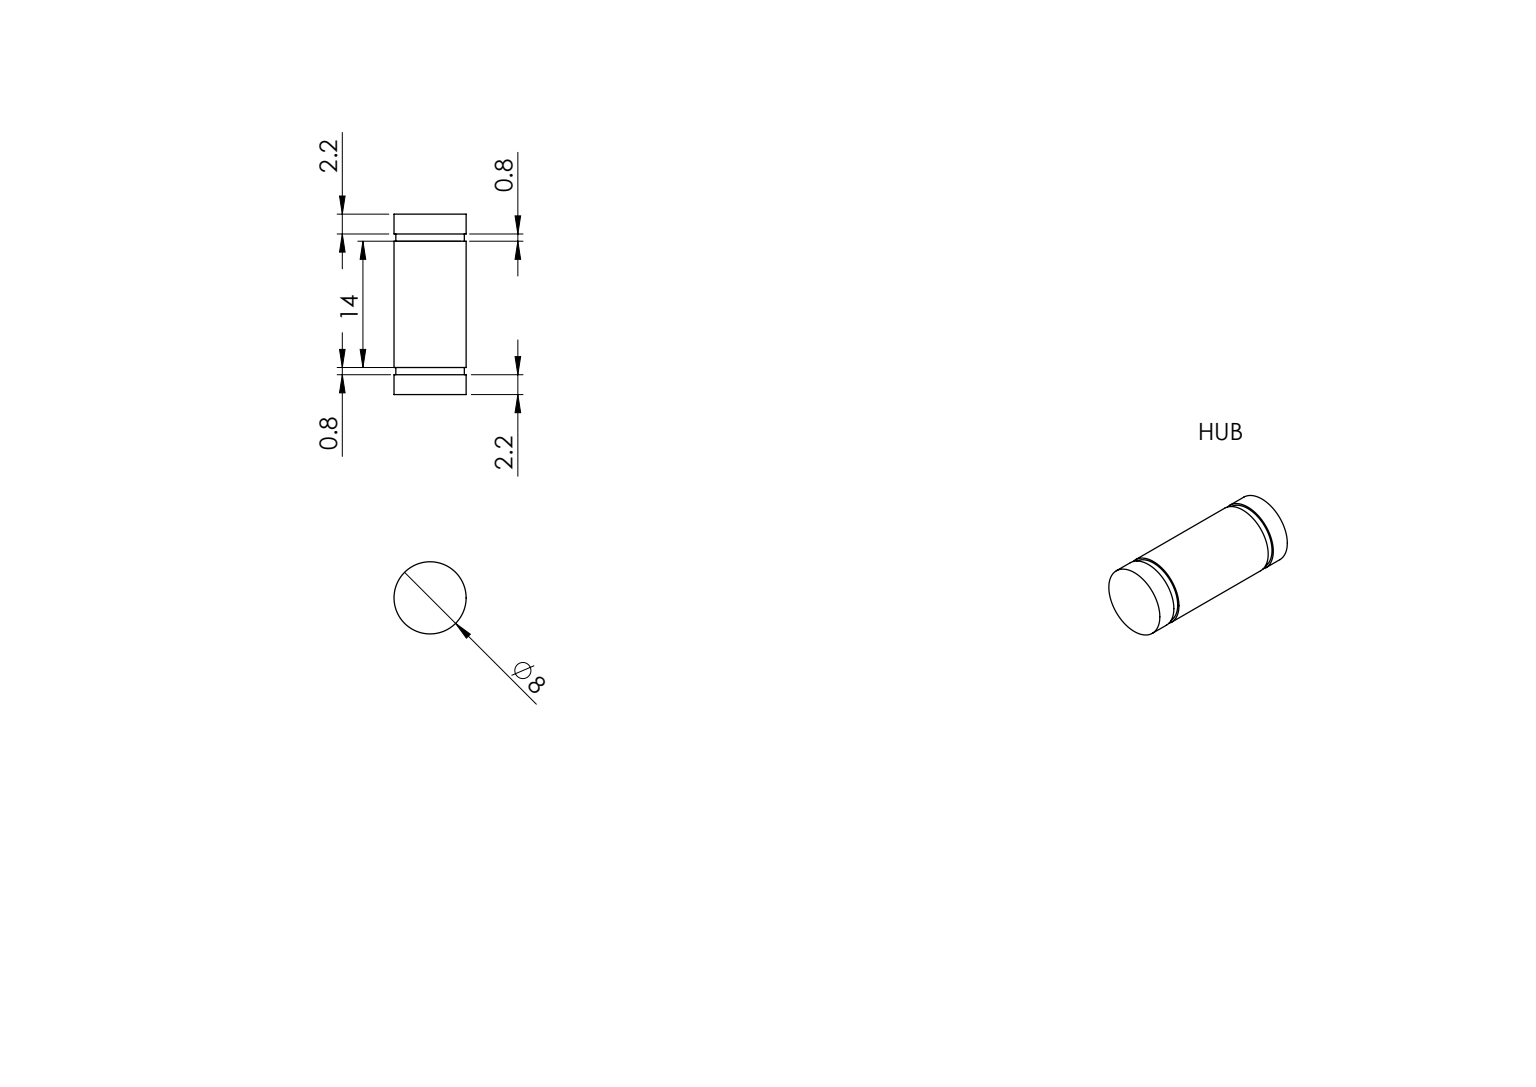
ISO-10303-21;
HEADER;
FILE_DESCRIPTION (('STEP AP214'),
    '1' );
FILE_NAME ('hub.step',
    '2026-10-31T03:41:51',
    ( '' ),
    ( '' ),
    'SwSTEP 2.0',
    'SolidWorks 2026',
    '' );
FILE_SCHEMA (( 'AUTOMOTIVE_DESIGN' ));
ENDSEC;

DATA;
#14=DIRECTION ( 'NONE',  ( -0.9873505073845697533, 0.1585527532634883052, 0.000000000000000000 ) ) ;
#15=CARTESIAN_POINT ( 'NONE',  ( 3.510166481118872639, 1.455586230640303791, -7.000000000000007994 ) ) ;
#136=FACE_BOUND ( 'NONE', #13544, .T. ) ;
#172=AXIS2_PLACEMENT_3D ( 'NONE', #5466, #3375, #833 ) ;
#177=ORIENTED_EDGE ( 'NONE', *, *, #10181, .F. ) ;
#188=VERTEX_POINT ( 'NONE', #5888 ) ;
#271=DIRECTION ( 'NONE',  ( -0.000000000000000000, -0.000000000000000000, -1.000000000000000000 ) ) ;
#281=AXIS2_PLACEMENT_3D ( 'NONE', #6195, #5139, #2580 ) ;
#334=EDGE_LOOP ( 'NONE', ( #5406, #2632 ) ) ;
#361=AXIS2_PLACEMENT_3D ( 'NONE', #2405, #5025, #1550 ) ;
#566=( NAMED_UNIT ( * ) SI_UNIT ( $, .STERADIAN. ) SOLID_ANGLE_UNIT ( ) );
#571=CLOSED_SHELL ( 'NONE', ( #13465, #1305, #9432, #9490, #3541, #14835, #4258, #10117, #4020, #1002, #1343, #9186, #11729, #8337, #8823, #13143 ) ) ;
#577=FACE_OUTER_BOUND ( 'NONE', #11814, .T. ) ;
#591=CIRCLE ( 'NONE', #1085, 3.799999999999999378 ) ;
#602=FACE_BOUND ( 'NONE', #4896, .T. ) ;
#684=ORIENTED_EDGE ( 'NONE', *, *, #14154, .F. ) ;
#686=CARTESIAN_POINT ( 'NONE',  ( 4.000000000000000888, 4.898587196589413815E-16, 10.00000000000000000 ) ) ;
#707=AXIS2_PLACEMENT_3D ( 'NONE', #4857, #13219, #9532 ) ;
#713=CYLINDRICAL_SURFACE ( 'NONE', #1338, 3.799999999999999378 ) ;
#813=CARTESIAN_POINT ( 'NONE',  ( -3.510166481118844661, -1.455586230640303347, -7.000000000000007994 ) ) ;
#833=DIRECTION ( 'NONE',  ( -1.000000000000000000, 0.000000000000000000, 0.000000000000000000 ) ) ;
#883=VERTEX_POINT ( 'NONE', #14448 ) ;
#897=CARTESIAN_POINT ( 'NONE',  ( 3.751931928061364552, -0.6025004624012525456, 7.799999999999990052 ) ) ;
#931=DIRECTION ( 'NONE',  ( 1.000000000000000000, 0.000000000000000000, 0.000000000000000000 ) ) ;
#943=CARTESIAN_POINT ( 'NONE',  ( 1.387778780781445676E-14, 0.000000000000000000, -7.800000000000008704 ) ) ;
#1002=ADVANCED_FACE ( 'NONE', ( #5726 ), #2188, .F. ) ;
#1012=CARTESIAN_POINT ( 'NONE',  ( 0.000000000000000000, 0.000000000000000000, -7.000000000000007994 ) ) ;
#1035=ORIENTED_EDGE ( 'NONE', *, *, #4321, .T. ) ;
#1080=DIRECTION ( 'NONE',  ( -5.339417856040273846E-17, -1.063174570779084847E-17, 1.000000000000000000 ) ) ;
#1085=AXIS2_PLACEMENT_3D ( 'NONE', #14018, #3483, #4499 ) ;
#1134=EDGE_CURVE ( 'NONE', #3521, #6501, #14102, .T. ) ;
#1157=CIRCLE ( 'NONE', #5838, 4.000000000000000888 ) ;
#1171=LINE ( 'NONE', #10842, #10236 ) ;
#1188=AXIS2_PLACEMENT_3D ( 'NONE', #7647, #14417, #6413 ) ;
#1211=EDGE_LOOP ( 'NONE', ( #2408, #10707 ) ) ;
#1233=EDGE_LOOP ( 'NONE', ( #2848, #13553 ) ) ;
#1243=DIRECTION ( 'NONE',  ( -0.000000000000000000, -0.000000000000000000, -1.000000000000000000 ) ) ;
#1305=ADVANCED_FACE ( 'NONE', ( #13545 ), #713, .T. ) ;
#1338=AXIS2_PLACEMENT_3D ( 'NONE', #9790, #10088, #14487 ) ;
#1343=ADVANCED_FACE ( 'NONE', ( #7786, #14944 ), #12543, .T. ) ;
#1376=AXIS2_PLACEMENT_3D ( 'NONE', #7353, #6187, #9640 ) ;
#1550=DIRECTION ( 'NONE',  ( -0.9873505073845698643, 0.1585527532634883330, -5.103307673902845341E-17 ) ) ;
#1569=EDGE_CURVE ( 'NONE', #883, #13931, #1171, .T. ) ;
#1595=CARTESIAN_POINT ( 'NONE',  ( 0.000000000000000000, 0.000000000000000000, 10.00000000000000000 ) ) ;
#1602=VECTOR ( 'NONE', #10196, 1000.000000000000000 ) ;
#1616=LINE ( 'NONE', #686, #9254 ) ;
#1694=DIRECTION ( 'NONE',  ( -5.339417856040273846E-17, -1.063174570779084847E-17, 1.000000000000000000 ) ) ;
#1753=EDGE_LOOP ( 'NONE', ( #13832, #7384, #14688, #11419 ) ) ;
#1802=( NAMED_UNIT ( * ) SI_UNIT ( $, .STERADIAN. ) SOLID_ANGLE_UNIT ( ) );
#1883=( LENGTH_UNIT ( ) NAMED_UNIT ( * ) SI_UNIT ( .MILLI., .METRE. ) );
#1912=CARTESIAN_POINT ( 'NONE',  ( 0.000000000000000000, 0.000000000000000000, 10.00000000000000000 ) ) ;
#1943=DIRECTION ( 'NONE',  ( -5.339417856040273846E-17, -1.063174570779084847E-17, 1.000000000000000000 ) ) ;
#1951=DIRECTION ( 'NONE',  ( -0.000000000000000000, 0.000000000000000000, -1.000000000000000000 ) ) ;
#2008=VERTEX_POINT ( 'NONE', #9753 ) ;
#2018=CARTESIAN_POINT ( 'NONE',  ( 1.387778780781445676E-14, 0.000000000000000000, -7.000000000000007994 ) ) ;
#2034=APPLICATION_CONTEXT ( 'automotive_design' ) ;
#2070=EDGE_CURVE ( 'NONE', #12014, #3521, #14593, .T. ) ;
#2083=FACE_OUTER_BOUND ( 'NONE', #4286, .T. ) ;
#2089=PRODUCT_DEFINITION_FORMATION_WITH_SPECIFIED_SOURCE ( 'ANY', '', #9463, .NOT_KNOWN. ) ;
#2101=CIRCLE ( 'NONE', #8723, 4.000000000000000888 ) ;
#2102=SURFACE_SIDE_STYLE ('',( #8863 ) ) ;
#2116=EDGE_CURVE ( 'NONE', #13784, #883, #8011, .T. ) ;
#2135=MECHANICAL_DESIGN_GEOMETRIC_PRESENTATION_REPRESENTATION('',(#3118),#5350);
#2171=CARTESIAN_POINT ( 'NONE',  ( 4.000000000000000888, 4.898587196589413815E-16, 10.00000000000000000 ) ) ;
#2179=AXIS2_PLACEMENT_3D ( 'NONE', #10380, #2241, #6855 ) ;
#2188=PLANE ( 'NONE',  #4532 ) ;
#2206=DIRECTION ( 'NONE',  ( 1.000000000000000000, 0.000000000000000000, 0.000000000000000000 ) ) ;
#2241=DIRECTION ( 'NONE',  ( 0.000000000000000000, 0.000000000000000000, -1.000000000000000000 ) ) ;
#2256=EDGE_LOOP ( 'NONE', ( #4202, #12754, #1035, #5511 ) ) ;
#2328=AXIS2_PLACEMENT_3D ( 'NONE', #7519, #12342, #12193 ) ;
#2380=AXIS2_PLACEMENT_3D ( 'NONE', #12215, #1694, #6377 ) ;
#2405=CARTESIAN_POINT ( 'NONE',  ( 0.000000000000000000, 3.361026734705063745E-15, 7.799999999999990052 ) ) ;
#2408=ORIENTED_EDGE ( 'NONE', *, *, #10953, .F. ) ;
#2414=CARTESIAN_POINT ( 'NONE',  ( -4.000000000000000888, 0.000000000000000000, 10.00000000000000000 ) ) ;
#2466=ORIENTED_EDGE ( 'NONE', *, *, #8770, .F. ) ;
#2512=EDGE_CURVE ( 'NONE', #12014, #2008, #6927, .T. ) ;
#2514=ORIENTED_EDGE ( 'NONE', *, *, #9096, .T. ) ;
#2517=FACE_OUTER_BOUND ( 'NONE', #8195, .T. ) ;
#2580=DIRECTION ( 'NONE',  ( -0.9873505073845697533, 0.1585527532634883052, 0.000000000000000000 ) ) ;
#2582=CIRCLE ( 'NONE', #6514, 3.799999999999999378 ) ;
#2632=ORIENTED_EDGE ( 'NONE', *, *, #6864, .T. ) ;
#2652=CIRCLE ( 'NONE', #14941, 4.000000000000000888 ) ;
#2658=LINE ( 'NONE', #6929, #4395 ) ;
#2743=EDGE_LOOP ( 'NONE', ( #6165, #4935, #6542, #7775 ) ) ;
#2819=CARTESIAN_POINT ( 'NONE',  ( -3.510166481118844661, -1.455586230640303347, -7.800000000000008704 ) ) ;
#2820=DIRECTION ( 'NONE',  ( -1.000000000000000000, 0.000000000000000000, 0.000000000000000000 ) ) ;
#2839=CYLINDRICAL_SURFACE ( 'NONE', #2380, 3.799999999999999378 ) ;
#2844=DIRECTION ( 'NONE',  ( 5.339417856040273846E-17, 1.063174570779084847E-17, -1.000000000000000000 ) ) ;
#2848=ORIENTED_EDGE ( 'NONE', *, *, #8770, .T. ) ;
#2906=PRODUCT_CONTEXT ( 'NONE', #2917, 'mechanical' ) ;
#2917=APPLICATION_CONTEXT ( 'automotive_design' ) ;
#2955=CARTESIAN_POINT ( 'NONE',  ( 3.510166481118872639, 1.455586230640303791, -7.000000000000007994 ) ) ;
#3031=PRESENTATION_STYLE_ASSIGNMENT (( #7803 ) ) ;
#3071=DIRECTION ( 'NONE',  ( 1.000000000000000000, 0.000000000000000000, 0.000000000000000000 ) ) ;
#3118=STYLED_ITEM('',(#15286),#3717);
#3147=CIRCLE ( 'NONE', #12705, 4.000000000000000888 ) ;
#3150=CARTESIAN_POINT ( 'NONE',  ( 3.751931928061364552, -0.6025004624012525456, 6.999999999999989342 ) ) ;
#3197=EDGE_CURVE ( 'NONE', #13784, #6657, #10149, .T. ) ;
#3243=ORIENTED_EDGE ( 'NONE', *, *, #7762, .F. ) ;
#3346=VERTEX_POINT ( 'NONE', #7605 ) ;
#3375=DIRECTION ( 'NONE',  ( -0.000000000000000000, -0.000000000000000000, -1.000000000000000000 ) ) ;
#3421=CARTESIAN_POINT ( 'NONE',  ( 0.000000000000000000, 0.000000000000000000, 10.00000000000000000 ) ) ;
#3483=DIRECTION ( 'NONE',  ( 5.339417856040273846E-17, 1.063174570779084847E-17, -1.000000000000000000 ) ) ;
#3501=ORIENTED_EDGE ( 'NONE', *, *, #3197, .T. ) ;
#3521=VERTEX_POINT ( 'NONE', #897 ) ;
#3541=ADVANCED_FACE ( 'NONE', ( #7749 ), #6821, .T. ) ;
#3551=CARTESIAN_POINT ( 'NONE',  ( 1.387778780781445676E-14, 0.000000000000000000, -7.000000000000007994 ) ) ;
#3604=AXIS2_PLACEMENT_3D ( 'NONE', #12463, #1080, #5778 ) ;
#3615=AXIS2_PLACEMENT_3D ( 'NONE', #5465, #4381, #3071 ) ;
#3618=AXIS2_PLACEMENT_3D ( 'NONE', #11876, #271, #10525 ) ;
#3630=DIRECTION ( 'NONE',  ( 0.000000000000000000, 0.000000000000000000, 1.000000000000000000 ) ) ;
#3717=MANIFOLD_SOLID_BREP ( 'Mirror2', #571 ) ;
#3797=CIRCLE ( 'NONE', #5048, 4.000000000000000888 ) ;
#3798=CYLINDRICAL_SURFACE ( 'NONE', #1188, 4.000000000000000888 ) ;
#3818=CARTESIAN_POINT ( 'NONE',  ( 0.000000000000000000, 0.000000000000000000, 7.799999999999990052 ) ) ;
#3932=CIRCLE ( 'NONE', #9806, 4.000000000000000888 ) ;
#3946=UNCERTAINTY_MEASURE_WITH_UNIT (LENGTH_MEASURE( 1.000000000000000082E-05 ), #1883, 'distance_accuracy_value', 'NONE');
#3986=DIRECTION ( 'NONE',  ( -1.000000000000000000, 0.000000000000000000, 0.000000000000000000 ) ) ;
#4020=ADVANCED_FACE ( 'NONE', ( #10493 ), #15108, .T. ) ;
#4202=ORIENTED_EDGE ( 'NONE', *, *, #11610, .F. ) ;
#4258=ADVANCED_FACE ( 'NONE', ( #11161 ), #7709, .T. ) ;
#4276=VERTEX_POINT ( 'NONE', #11317 ) ;
#4286=EDGE_LOOP ( 'NONE', ( #12799, #3243, #14483, #11996 ) ) ;
#4300=CYLINDRICAL_SURFACE ( 'NONE', #172, 4.000000000000000888 ) ;
#4321=EDGE_CURVE ( 'NONE', #10385, #9762, #9622, .T. ) ;
#4381=DIRECTION ( 'NONE',  ( -5.339417856040273846E-17, -1.063174570779084847E-17, 1.000000000000000000 ) ) ;
#4395=VECTOR ( 'NONE', #8941, 1000.000000000000000 ) ;
#4499=DIRECTION ( 'NONE',  ( -0.9873505073845697533, 0.1585527532634883052, 0.000000000000000000 ) ) ;
#4532=AXIS2_PLACEMENT_3D ( 'NONE', #14674, #8966, #9974 ) ;
#4583=( GEOMETRIC_REPRESENTATION_CONTEXT ( 3 ) GLOBAL_UNCERTAINTY_ASSIGNED_CONTEXT ( ( #3946 ) ) GLOBAL_UNIT_ASSIGNED_CONTEXT ( ( #1883, #12487, #10101 ) ) REPRESENTATION_CONTEXT ( 'NONE', 'WORKASPACE' ) );
#4633=ORIENTED_EDGE ( 'NONE', *, *, #14894, .T. ) ;
#4673=DIRECTION ( 'NONE',  ( -0.9237280213470681067, -0.3830490080632377725, 0.000000000000000000 ) ) ;
#4700=ORIENTED_EDGE ( 'NONE', *, *, #1134, .F. ) ;
#4722=ORIENTED_EDGE ( 'NONE', *, *, #8548, .F. ) ;
#4857=CARTESIAN_POINT ( 'NONE',  ( 1.387778780781445676E-14, 0.000000000000000000, -7.800000000000008704 ) ) ;
#4871=ORIENTED_EDGE ( 'NONE', *, *, #6559, .T. ) ;
#4896=EDGE_LOOP ( 'NONE', ( #14625, #8838 ) ) ;
#4935=ORIENTED_EDGE ( 'NONE', *, *, #2070, .T. ) ;
#4954=CARTESIAN_POINT ( 'NONE',  ( 4.000000000000000888, 4.898587196589413815E-16, -10.00000000000000000 ) ) ;
#5025=DIRECTION ( 'NONE',  ( -5.339417856040274462E-17, -1.063174570779084693E-17, 1.000000000000000000 ) ) ;
#5048=AXIS2_PLACEMENT_3D ( 'NONE', #1595, #5741, #2206 ) ;
#5139=DIRECTION ( 'NONE',  ( 5.339417856040273846E-17, 1.063174570779084847E-17, -1.000000000000000000 ) ) ;
#5164=ORIENTED_EDGE ( 'NONE', *, *, #5328, .F. ) ;
#5180=ORIENTED_EDGE ( 'NONE', *, *, #10953, .T. ) ;
#5220=CARTESIAN_POINT ( 'NONE',  ( 0.000000000000000000, 0.000000000000000000, 10.00000000000000000 ) ) ;
#5271=CARTESIAN_POINT ( 'NONE',  ( 4.000000000000000888, 4.898587196589413815E-16, 6.999999999999989342 ) ) ;
#5283=VECTOR ( 'NONE', #8994, 1000.000000000000000 ) ;
#5292=AXIS2_PLACEMENT_3D ( 'NONE', #10991, #2844, #12130 ) ;
#5296=CYLINDRICAL_SURFACE ( 'NONE', #14910, 4.000000000000000888 ) ;
#5316=AXIS2_PLACEMENT_3D ( 'NONE', #12069, #11998, #8688 ) ;
#5321=PLANE ( 'NONE',  #14351 ) ;
#5328=EDGE_CURVE ( 'NONE', #14141, #11359, #3932, .T. ) ;
#5333=VERTEX_POINT ( 'NONE', #13616 ) ;
#5350=( GEOMETRIC_REPRESENTATION_CONTEXT ( 3 ) GLOBAL_UNCERTAINTY_ASSIGNED_CONTEXT ( ( #13840 ) ) GLOBAL_UNIT_ASSIGNED_CONTEXT ( ( #6421, #11104, #566 ) ) REPRESENTATION_CONTEXT ( 'NONE', 'WORKASPACE' ) );
#5406=ORIENTED_EDGE ( 'NONE', *, *, #11003, .T. ) ;
#5412=EDGE_LOOP ( 'NONE', ( #684, #14580, #13715, #9552 ) ) ;
#5465=CARTESIAN_POINT ( 'NONE',  ( 0.000000000000000000, 0.000000000000000000, 6.999999999999989342 ) ) ;
#5466=CARTESIAN_POINT ( 'NONE',  ( 0.000000000000000000, 0.000000000000000000, 10.00000000000000000 ) ) ;
#5469=CARTESIAN_POINT ( 'NONE',  ( 4.271534284832219323E-17, 3.369532131271296443E-15, 6.999999999999989342 ) ) ;
#5500=SHAPE_REPRESENTATION_RELATIONSHIP ( 'NONE' , 'NONE' ,  #5737, #14983 ) ;
#5511=ORIENTED_EDGE ( 'NONE', *, *, #11130, .F. ) ;
#5567=DIRECTION ( 'NONE',  ( -0.000000000000000000, -0.000000000000000000, -1.000000000000000000 ) ) ;
#5580=AXIS2_PLACEMENT_3D ( 'NONE', #1912, #10350, #6604 ) ;
#5650=EDGE_LOOP ( 'NONE', ( #5180, #3501, #4633, #6543 ) ) ;
#5726=FACE_OUTER_BOUND ( 'NONE', #7587, .T. ) ;
#5737=SHAPE_REPRESENTATION ( 'hub', ( #1376 ), #12207 ) ;
#5741=DIRECTION ( 'NONE',  ( 0.000000000000000000, 0.000000000000000000, 1.000000000000000000 ) ) ;
#5778=DIRECTION ( 'NONE',  ( -0.9873505073845697533, 0.1585527532634883052, 0.000000000000000000 ) ) ;
#5805=VECTOR ( 'NONE', #14677, 1000.000000000000000 ) ;
#5838=AXIS2_PLACEMENT_3D ( 'NONE', #10962, #13505, #7662 ) ;
#5888=CARTESIAN_POINT ( 'NONE',  ( -4.000000000000000888, 0.000000000000000000, 10.00000000000000000 ) ) ;
#5946=DIRECTION ( 'NONE',  ( -0.000000000000000000, -0.000000000000000000, -1.000000000000000000 ) ) ;
#5953=AXIS2_PLACEMENT_3D ( 'NONE', #943, #12395, #10321 ) ;
#6018=CIRCLE ( 'NONE', #12873, 3.799999999999999378 ) ;
#6069=CIRCLE ( 'NONE', #7550, 4.000000000000000888 ) ;
#6091=DIRECTION ( 'NONE',  ( 1.000000000000000000, 0.000000000000000000, 0.000000000000000000 ) ) ;
#6162=CARTESIAN_POINT ( 'NONE',  ( 0.000000000000000000, 0.000000000000000000, -10.00000000000000000 ) ) ;
#6165=ORIENTED_EDGE ( 'NONE', *, *, #2512, .F. ) ;
#6187=DIRECTION ( 'NONE',  ( 0.000000000000000000, 0.000000000000000000, 1.000000000000000000 ) ) ;
#6195=CARTESIAN_POINT ( 'NONE',  ( 4.271534284832219323E-17, 3.369532131271296443E-15, 6.999999999999989342 ) ) ;
#6203=ORIENTED_EDGE ( 'NONE', *, *, #14886, .F. ) ;
#6235=FACE_BOUND ( 'NONE', #13768, .T. ) ;
#6294=ORIENTED_EDGE ( 'NONE', *, *, #5328, .T. ) ;
#6377=DIRECTION ( 'NONE',  ( -0.9873505073845697533, 0.1585527532634883052, 0.000000000000000000 ) ) ;
#6413=DIRECTION ( 'NONE',  ( -1.000000000000000000, 0.000000000000000000, 0.000000000000000000 ) ) ;
#6421=( LENGTH_UNIT ( ) NAMED_UNIT ( * ) SI_UNIT ( .MILLI., .METRE. ) );
#6501=VERTEX_POINT ( 'NONE', #11698 ) ;
#6514=AXIS2_PLACEMENT_3D ( 'NONE', #3551, #3630, #8320 ) ;
#6540=VERTEX_POINT ( 'NONE', #15 ) ;
#6542=ORIENTED_EDGE ( 'NONE', *, *, #1134, .T. ) ;
#6543=ORIENTED_EDGE ( 'NONE', *, *, #1569, .F. ) ;
#6559=EDGE_CURVE ( 'NONE', #188, #3346, #15029, .T. ) ;
#6562=CARTESIAN_POINT ( 'NONE',  ( 0.000000000000000000, 0.000000000000000000, 10.00000000000000000 ) ) ;
#6604=DIRECTION ( 'NONE',  ( -1.000000000000000000, 0.000000000000000000, 0.000000000000000000 ) ) ;
#6657=VERTEX_POINT ( 'NONE', #4954 ) ;
#6693=CARTESIAN_POINT ( 'NONE',  ( 4.000000000000000888, 4.898587196589413815E-16, 10.00000000000000000 ) ) ;
#6744=CIRCLE ( 'NONE', #2328, 4.000000000000000888 ) ;
#6747=AXIS2_PLACEMENT_3D ( 'NONE', #13065, #7251, #14 ) ;
#6793=( NAMED_UNIT ( * ) PLANE_ANGLE_UNIT ( ) SI_UNIT ( $, .RADIAN. ) );
#6814=AXIS2_PLACEMENT_3D ( 'NONE', #9407, #14261, #4673 ) ;
#6821=CYLINDRICAL_SURFACE ( 'NONE', #5580, 4.000000000000000888 ) ;
#6855=DIRECTION ( 'NONE',  ( -1.000000000000000000, 0.000000000000000000, 0.000000000000000000 ) ) ;
#6856=DIRECTION ( 'NONE',  ( -0.000000000000000000, -0.000000000000000000, -1.000000000000000000 ) ) ;
#6864=EDGE_CURVE ( 'NONE', #5333, #188, #2652, .T. ) ;
#6927=CIRCLE ( 'NONE', #281, 3.799999999999999378 ) ;
#6929=CARTESIAN_POINT ( 'NONE',  ( -4.000000000000000888, 0.000000000000000000, 10.00000000000000000 ) ) ;
#7055=CIRCLE ( 'NONE', #6814, 3.799999999999999378 ) ;
#7162=ORIENTED_EDGE ( 'NONE', *, *, #12918, .F. ) ;
#7251=DIRECTION ( 'NONE',  ( 5.339417856040273846E-17, 1.063174570779084847E-17, -1.000000000000000000 ) ) ;
#7280=EDGE_LOOP ( 'NONE', ( #6203, #11454 ) ) ;
#7283=CYLINDRICAL_SURFACE ( 'NONE', #3618, 4.000000000000000888 ) ;
#7334=CYLINDRICAL_SURFACE ( 'NONE', #5316, 3.799999999999999378 ) ;
#7353=CARTESIAN_POINT ( 'NONE',  ( 0.000000000000000000, 0.000000000000000000, 0.000000000000000000 ) ) ;
#7384=ORIENTED_EDGE ( 'NONE', *, *, #2116, .T. ) ;
#7403=PLANE ( 'NONE',  #361 ) ;
#7496=CARTESIAN_POINT ( 'NONE',  ( -4.000000000000000888, 0.000000000000000000, -7.000000000000007994 ) ) ;
#7518=DIRECTION ( 'NONE',  ( -5.339417856040273846E-17, -1.063174570779084847E-17, 1.000000000000000000 ) ) ;
#7519=CARTESIAN_POINT ( 'NONE',  ( 0.000000000000000000, 0.000000000000000000, -7.800000000000010481 ) ) ;
#7531=ORIENTED_EDGE ( 'NONE', *, *, #14259, .T. ) ;
#7550=AXIS2_PLACEMENT_3D ( 'NONE', #3818, #7518, #14516 ) ;
#7558=STYLED_ITEM ( 'NONE', ( #3031 ), #14983 ) ;
#7587=EDGE_LOOP ( 'NONE', ( #7162, #14662 ) ) ;
#7605=CARTESIAN_POINT ( 'NONE',  ( -4.000000000000000888, 2.270693314922320170E-33, 7.799999999999990052 ) ) ;
#7647=CARTESIAN_POINT ( 'NONE',  ( 0.000000000000000000, 0.000000000000000000, 10.00000000000000000 ) ) ;
#7662=DIRECTION ( 'NONE',  ( 1.000000000000000000, 0.000000000000000000, 0.000000000000000000 ) ) ;
#7709=CYLINDRICAL_SURFACE ( 'NONE', #10365, 4.000000000000000888 ) ;
#7749=FACE_OUTER_BOUND ( 'NONE', #14904, .T. ) ;
#7762=EDGE_CURVE ( 'NONE', #2008, #12014, #591, .T. ) ;
#7771=PRODUCT_DEFINITION ( 'UNKNOWN', '', #2089, #13466 ) ;
#7775=ORIENTED_EDGE ( 'NONE', *, *, #8037, .F. ) ;
#7786=FACE_BOUND ( 'NONE', #1233, .T. ) ;
#7789=CARTESIAN_POINT ( 'NONE',  ( -3.751931928061364552, 0.6025004624012588739, 6.999999999999989342 ) ) ;
#7803=SURFACE_STYLE_USAGE ( .BOTH. , #2102 ) ;
#7869=CARTESIAN_POINT ( 'NONE',  ( -4.000000000000000888, 2.270693314922320170E-33, 6.999999999999989342 ) ) ;
#7908=CARTESIAN_POINT ( 'NONE',  ( -3.510166481118844661, -1.455586230640303347, -7.000000000000007994 ) ) ;
#7928=CYLINDRICAL_SURFACE ( 'NONE', #3604, 3.799999999999999378 ) ;
#7930=CARTESIAN_POINT ( 'NONE',  ( 0.000000000000000000, 0.000000000000000000, 7.799999999999990052 ) ) ;
#7934=DIRECTION ( 'NONE',  ( -0.9237280213470682178, -0.3830490080632377725, 0.000000000000000000 ) ) ;
#7983=VERTEX_POINT ( 'NONE', #7869 ) ;
#8011=CIRCLE ( 'NONE', #12169, 4.000000000000000888 ) ;
#8037=EDGE_CURVE ( 'NONE', #2008, #6501, #10164, .T. ) ;
#8155=EDGE_LOOP ( 'NONE', ( #4722, #2466, #9128, #15107 ) ) ;
#8167=AXIS2_PLACEMENT_3D ( 'NONE', #3421, #11781, #9400 ) ;
#8169=EDGE_CURVE ( 'NONE', #6501, #3521, #8449, .T. ) ;
#8195=EDGE_LOOP ( 'NONE', ( #11263, #12072, #5164, #177 ) ) ;
#8320=DIRECTION ( 'NONE',  ( -0.9237280213470681067, -0.3830490080632377725, 0.000000000000000000 ) ) ;
#8337=ADVANCED_FACE ( 'NONE', ( #602, #8907 ), #5321, .T. ) ;
#8378=DIRECTION ( 'NONE',  ( 0.000000000000000000, 0.000000000000000000, 1.000000000000000000 ) ) ;
#8449=CIRCLE ( 'NONE', #5292, 3.799999999999999378 ) ;
#8528=PLANE ( 'NONE',  #707 ) ;
#8545=FACE_OUTER_BOUND ( 'NONE', #7280, .T. ) ;
#8548=EDGE_CURVE ( 'NONE', #6540, #10385, #14791, .T. ) ;
#8556=VECTOR ( 'NONE', #5946, 1000.000000000000000 ) ;
#8585=DIRECTION ( 'NONE',  ( -0.000000000000000000, -0.000000000000000000, -1.000000000000000000 ) ) ;
#8688=DIRECTION ( 'NONE',  ( -0.9237280213470681067, -0.3830490080632377725, 0.000000000000000000 ) ) ;
#8693=CARTESIAN_POINT ( 'NONE',  ( 0.000000000000000000, 0.000000000000000000, 10.00000000000000000 ) ) ;
#8723=AXIS2_PLACEMENT_3D ( 'NONE', #6162, #8378, #6091 ) ;
#8770=EDGE_CURVE ( 'NONE', #11997, #6540, #6018, .T. ) ;
#8823=ADVANCED_FACE ( 'NONE', ( #8545, #6235 ), #7403, .F. ) ;
#8838=ORIENTED_EDGE ( 'NONE', *, *, #2512, .T. ) ;
#8854=DIRECTION ( 'NONE',  ( -5.339417856040273846E-17, -1.063174570779084847E-17, 1.000000000000000000 ) ) ;
#8863=SURFACE_STYLE_FILL_AREA ( #11324 ) ;
#8907=FACE_OUTER_BOUND ( 'NONE', #11914, .T. ) ;
#8941=DIRECTION ( 'NONE',  ( -0.000000000000000000, -0.000000000000000000, -1.000000000000000000 ) ) ;
#8966=DIRECTION ( 'NONE',  ( 0.000000000000000000, 0.000000000000000000, 1.000000000000000000 ) ) ;
#8994=DIRECTION ( 'NONE',  ( -0.000000000000000000, -0.000000000000000000, -1.000000000000000000 ) ) ;
#9031=VECTOR ( 'NONE', #6856, 1000.000000000000000 ) ;
#9038=ORIENTED_EDGE ( 'NONE', *, *, #11003, .F. ) ;
#9088=DIRECTION ( 'NONE',  ( -5.339417856040273846E-17, -1.063174570779084847E-17, 1.000000000000000000 ) ) ;
#9096=EDGE_CURVE ( 'NONE', #11359, #14141, #11463, .T. ) ;
#9128=ORIENTED_EDGE ( 'NONE', *, *, #11130, .T. ) ;
#9186=ADVANCED_FACE ( 'NONE', ( #10684, #136 ), #8528, .F. ) ;
#9253=ORIENTED_EDGE ( 'NONE', *, *, #6864, .F. ) ;
#9254=VECTOR ( 'NONE', #12358, 1000.000000000000000 ) ;
#9327=CARTESIAN_POINT ( 'NONE',  ( 1.387778780781445676E-14, 0.000000000000000000, -7.000000000000007994 ) ) ;
#9400=DIRECTION ( 'NONE',  ( 1.000000000000000000, 0.000000000000000000, -0.000000000000000000 ) ) ;
#9407=CARTESIAN_POINT ( 'NONE',  ( 1.387778780781445676E-14, 0.000000000000000000, -7.800000000000008704 ) ) ;
#9432=ADVANCED_FACE ( 'NONE', ( #15058 ), #4300, .T. ) ;
#9463=PRODUCT ( 'hub', 'hub', '', ( #2906 ) ) ;
#9490=ADVANCED_FACE ( 'NONE', ( #2517 ), #7283, .T. ) ;
#9532=DIRECTION ( 'NONE',  ( -0.9237280213470682178, -0.3830490080632377725, 0.000000000000000000 ) ) ;
#9552=ORIENTED_EDGE ( 'NONE', *, *, #9096, .F. ) ;
#9622=CIRCLE ( 'NONE', #5953, 3.799999999999999378 ) ;
#9640=DIRECTION ( 'NONE',  ( 1.000000000000000000, 0.000000000000000000, 0.000000000000000000 ) ) ;
#9753=CARTESIAN_POINT ( 'NONE',  ( -3.751931928061364552, 0.6025004624012588739, 6.999999999999989342 ) ) ;
#9762=VERTEX_POINT ( 'NONE', #2819 ) ;
#9790=CARTESIAN_POINT ( 'NONE',  ( 1.387778780781445676E-14, 0.000000000000000000, -7.000000000000007994 ) ) ;
#9806=AXIS2_PLACEMENT_3D ( 'NONE', #1012, #10384, #15081 ) ;
#9817=ORIENTED_EDGE ( 'NONE', *, *, #15097, .F. ) ;
#9869=FACE_OUTER_BOUND ( 'NONE', #1753, .T. ) ;
#9887=SHAPE_DEFINITION_REPRESENTATION ( #11545, #5737 ) ;
#9974=DIRECTION ( 'NONE',  ( 1.000000000000000000, 0.000000000000000000, -0.000000000000000000 ) ) ;
#9991=DIRECTION ( 'NONE',  ( -5.339417856040274462E-17, -1.063174570779084693E-17, 1.000000000000000000 ) ) ;
#10088=DIRECTION ( 'NONE',  ( 0.000000000000000000, 0.000000000000000000, -1.000000000000000000 ) ) ;
#10101=( NAMED_UNIT ( * ) SI_UNIT ( $, .STERADIAN. ) SOLID_ANGLE_UNIT ( ) );
#10117=ADVANCED_FACE ( 'NONE', ( #9869 ), #3798, .T. ) ;
#10149=LINE ( 'NONE', #6693, #5283 ) ;
#10164=LINE ( 'NONE', #7789, #14337 ) ;
#10176=AXIS2_PLACEMENT_3D ( 'NONE', #2018, #1951, #7934 ) ;
#10181=EDGE_CURVE ( 'NONE', #7983, #14141, #2658, .T. ) ;
#10196=DIRECTION ( 'NONE',  ( 0.000000000000000000, 0.000000000000000000, -1.000000000000000000 ) ) ;
#10236=VECTOR ( 'NONE', #1243, 1000.000000000000000 ) ;
#10321=DIRECTION ( 'NONE',  ( -0.9237280213470681067, -0.3830490080632377725, 0.000000000000000000 ) ) ;
#10350=DIRECTION ( 'NONE',  ( -0.000000000000000000, -0.000000000000000000, -1.000000000000000000 ) ) ;
#10365=AXIS2_PLACEMENT_3D ( 'NONE', #6562, #5567, #13625 ) ;
#10380=CARTESIAN_POINT ( 'NONE',  ( 0.000000000000000000, 0.000000000000000000, -7.000000000000007994 ) ) ;
#10384=DIRECTION ( 'NONE',  ( 0.000000000000000000, 0.000000000000000000, -1.000000000000000000 ) ) ;
#10385=VERTEX_POINT ( 'NONE', #14383 ) ;
#10493=FACE_OUTER_BOUND ( 'NONE', #334, .T. ) ;
#10525=DIRECTION ( 'NONE',  ( -1.000000000000000000, 0.000000000000000000, 0.000000000000000000 ) ) ;
#10672=VECTOR ( 'NONE', #11320, 1000.000000000000000 ) ;
#10684=FACE_OUTER_BOUND ( 'NONE', #1211, .T. ) ;
#10707=ORIENTED_EDGE ( 'NONE', *, *, #2116, .F. ) ;
#10842=CARTESIAN_POINT ( 'NONE',  ( -4.000000000000000888, 0.000000000000000000, 10.00000000000000000 ) ) ;
#10845=ORIENTED_EDGE ( 'NONE', *, *, #8169, .F. ) ;
#10895=CARTESIAN_POINT ( 'NONE',  ( 0.000000000000000000, 0.000000000000000000, -7.800000000000010481 ) ) ;
#10947=ORIENTED_EDGE ( 'NONE', *, *, #14886, .T. ) ;
#10953=EDGE_CURVE ( 'NONE', #883, #13784, #6744, .T. ) ;
#10955=ORIENTED_EDGE ( 'NONE', *, *, #13199, .T. ) ;
#10962=CARTESIAN_POINT ( 'NONE',  ( 0.000000000000000000, 0.000000000000000000, -10.00000000000000000 ) ) ;
#10991=CARTESIAN_POINT ( 'NONE',  ( 0.000000000000000000, 3.361026734705063745E-15, 7.799999999999990052 ) ) ;
#11003=EDGE_CURVE ( 'NONE', #188, #5333, #3797, .T. ) ;
#11082=FACE_OUTER_BOUND ( 'NONE', #8155, .T. ) ;
#11104=( NAMED_UNIT ( * ) PLANE_ANGLE_UNIT ( ) SI_UNIT ( $, .RADIAN. ) );
#11130=EDGE_CURVE ( 'NONE', #11997, #9762, #12509, .T. ) ;
#11161=FACE_OUTER_BOUND ( 'NONE', #5412, .T. ) ;
#11168=ORIENTED_EDGE ( 'NONE', *, *, #13422, .F. ) ;
#11263=ORIENTED_EDGE ( 'NONE', *, *, #13199, .F. ) ;
#11317=CARTESIAN_POINT ( 'NONE',  ( 4.000000000000000888, 4.898587196589413815E-16, 7.799999999999990052 ) ) ;
#11320=DIRECTION ( 'NONE',  ( 0.000000000000000000, 0.000000000000000000, -1.000000000000000000 ) ) ;
#11324=FILL_AREA_STYLE ('',( #13558 ) ) ;
#11359=VERTEX_POINT ( 'NONE', #13488 ) ;
#11375=ORIENTED_EDGE ( 'NONE', *, *, #4321, .F. ) ;
#11419=ORIENTED_EDGE ( 'NONE', *, *, #12918, .T. ) ;
#11454=ORIENTED_EDGE ( 'NONE', *, *, #14259, .F. ) ;
#11463=CIRCLE ( 'NONE', #2179, 4.000000000000000888 ) ;
#11465=DIRECTION ( 'NONE',  ( 1.000000000000000000, 0.000000000000000000, 0.000000000000000000 ) ) ;
#11470=MECHANICAL_DESIGN_GEOMETRIC_PRESENTATION_REPRESENTATION('',(#7558),#4583);
#11545=PRODUCT_DEFINITION_SHAPE ( 'NONE', 'NONE',  #7771 ) ;
#11610=EDGE_CURVE ( 'NONE', #6540, #11997, #2582, .T. ) ;
#11698=CARTESIAN_POINT ( 'NONE',  ( -3.751931928061364552, 0.6025004624012588739, 7.799999999999990052 ) ) ;
#11729=ADVANCED_FACE ( 'NONE', ( #11082 ), #7334, .T. ) ;
#11781=DIRECTION ( 'NONE',  ( 0.000000000000000000, 0.000000000000000000, 1.000000000000000000 ) ) ;
#11814=EDGE_LOOP ( 'NONE', ( #11168, #9038, #4871, #10947 ) ) ;
#11876=CARTESIAN_POINT ( 'NONE',  ( 0.000000000000000000, 0.000000000000000000, 10.00000000000000000 ) ) ;
#11914=EDGE_LOOP ( 'NONE', ( #14867, #10955 ) ) ;
#11995=DIRECTION ( 'NONE',  ( 0.000000000000000000, 0.000000000000000000, 1.000000000000000000 ) ) ;
#11996=ORIENTED_EDGE ( 'NONE', *, *, #8169, .T. ) ;
#11997=VERTEX_POINT ( 'NONE', #7908 ) ;
#11998=DIRECTION ( 'NONE',  ( 0.000000000000000000, 0.000000000000000000, -1.000000000000000000 ) ) ;
#12014=VERTEX_POINT ( 'NONE', #3150 ) ;
#12068=UNCERTAINTY_MEASURE_WITH_UNIT (LENGTH_MEASURE( 1.000000000000000082E-05 ), #12555, 'distance_accuracy_value', 'NONE');
#12069=CARTESIAN_POINT ( 'NONE',  ( 1.387778780781445676E-14, 0.000000000000000000, -7.000000000000007994 ) ) ;
#12072=ORIENTED_EDGE ( 'NONE', *, *, #14154, .T. ) ;
#12130=DIRECTION ( 'NONE',  ( -0.9873505073845697533, 0.1585527532634883052, 0.000000000000000000 ) ) ;
#12165=LINE ( 'NONE', #2171, #9031 ) ;
#12169=AXIS2_PLACEMENT_3D ( 'NONE', #10895, #13205, #3986 ) ;
#12191=CIRCLE ( 'NONE', #13164, 4.000000000000000888 ) ;
#12193=DIRECTION ( 'NONE',  ( -1.000000000000000000, 0.000000000000000000, 0.000000000000000000 ) ) ;
#12207=( GEOMETRIC_REPRESENTATION_CONTEXT ( 3 ) GLOBAL_UNCERTAINTY_ASSIGNED_CONTEXT ( ( #12068 ) ) GLOBAL_UNIT_ASSIGNED_CONTEXT ( ( #12555, #6793, #1802 ) ) REPRESENTATION_CONTEXT ( 'NONE', 'WORKASPACE' ) );
#12215=CARTESIAN_POINT ( 'NONE',  ( 4.271534284832219323E-17, 3.369532131271296443E-15, 6.999999999999989342 ) ) ;
#12282=CARTESIAN_POINT ( 'NONE',  ( 3.751931928061364552, -0.6025004624012525456, 6.999999999999989342 ) ) ;
#12342=DIRECTION ( 'NONE',  ( 0.000000000000000000, 0.000000000000000000, -1.000000000000000000 ) ) ;
#12358=DIRECTION ( 'NONE',  ( -0.000000000000000000, -0.000000000000000000, -1.000000000000000000 ) ) ;
#12395=DIRECTION ( 'NONE',  ( 0.000000000000000000, 0.000000000000000000, 1.000000000000000000 ) ) ;
#12463=CARTESIAN_POINT ( 'NONE',  ( 4.271534284832219323E-17, 3.369532131271296443E-15, 6.999999999999989342 ) ) ;
#12487=( NAMED_UNIT ( * ) PLANE_ANGLE_UNIT ( ) SI_UNIT ( $, .RADIAN. ) );
#12509=LINE ( 'NONE', #813, #1602 ) ;
#12543=PLANE ( 'NONE',  #10176 ) ;
#12555=( LENGTH_UNIT ( ) NAMED_UNIT ( * ) SI_UNIT ( .MILLI., .METRE. ) );
#12618=VERTEX_POINT ( 'NONE', #5271 ) ;
#12705=AXIS2_PLACEMENT_3D ( 'NONE', #7930, #9088, #13772 ) ;
#12754=ORIENTED_EDGE ( 'NONE', *, *, #8548, .T. ) ;
#12799=ORIENTED_EDGE ( 'NONE', *, *, #2070, .F. ) ;
#12873=AXIS2_PLACEMENT_3D ( 'NONE', #9327, #11995, #14077 ) ;
#12918=EDGE_CURVE ( 'NONE', #13931, #6657, #2101, .T. ) ;
#13065=CARTESIAN_POINT ( 'NONE',  ( 0.000000000000000000, 3.361026734705063745E-15, 7.799999999999990052 ) ) ;
#13143=ADVANCED_FACE ( 'NONE', ( #2083 ), #7928, .T. ) ;
#13164=AXIS2_PLACEMENT_3D ( 'NONE', #15074, #1943, #931 ) ;
#13199=EDGE_CURVE ( 'NONE', #12618, #7983, #12191, .T. ) ;
#13205=DIRECTION ( 'NONE',  ( 0.000000000000000000, 0.000000000000000000, -1.000000000000000000 ) ) ;
#13219=DIRECTION ( 'NONE',  ( -0.000000000000000000, 0.000000000000000000, -1.000000000000000000 ) ) ;
#13338=CARTESIAN_POINT ( 'NONE',  ( 4.000000000000000888, 4.898587196589413815E-16, -7.800000000000010481 ) ) ;
#13360=FACE_OUTER_BOUND ( 'NONE', #2743, .T. ) ;
#13422=EDGE_CURVE ( 'NONE', #5333, #4276, #1616, .T. ) ;
#13465=ADVANCED_FACE ( 'NONE', ( #13360 ), #2839, .T. ) ;
#13466=PRODUCT_DEFINITION_CONTEXT ( 'detailed design', #2034, 'design' ) ;
#13488=CARTESIAN_POINT ( 'NONE',  ( 4.000000000000000888, 4.898587196589413815E-16, -7.000000000000007994 ) ) ;
#13505=DIRECTION ( 'NONE',  ( 0.000000000000000000, 0.000000000000000000, 1.000000000000000000 ) ) ;
#13512=EDGE_CURVE ( 'NONE', #7983, #12618, #14174, .T. ) ;
#13544=EDGE_LOOP ( 'NONE', ( #9817, #11375 ) ) ;
#13545=FACE_OUTER_BOUND ( 'NONE', #2256, .T. ) ;
#13553=ORIENTED_EDGE ( 'NONE', *, *, #11610, .T. ) ;
#13558=FILL_AREA_STYLE_COLOUR ( '', #14176 ) ;
#13616=CARTESIAN_POINT ( 'NONE',  ( 4.000000000000000888, 4.898587196589413815E-16, 10.00000000000000000 ) ) ;
#13625=DIRECTION ( 'NONE',  ( -1.000000000000000000, 0.000000000000000000, 0.000000000000000000 ) ) ;
#13715=ORIENTED_EDGE ( 'NONE', *, *, #10181, .T. ) ;
#13753=EDGE_LOOP ( 'NONE', ( #6294, #2514 ) ) ;
#13757=DIRECTION ( 'NONE',  ( -0.9873505073845698643, 0.1585527532634883330, -5.103307673902845341E-17 ) ) ;
#13768=EDGE_LOOP ( 'NONE', ( #10845, #4700 ) ) ;
#13772=DIRECTION ( 'NONE',  ( 1.000000000000000000, 0.000000000000000000, 0.000000000000000000 ) ) ;
#13784=VERTEX_POINT ( 'NONE', #13338 ) ;
#13832=ORIENTED_EDGE ( 'NONE', *, *, #3197, .F. ) ;
#13840=UNCERTAINTY_MEASURE_WITH_UNIT (LENGTH_MEASURE( 1.000000000000000082E-05 ), #6421, 'distance_accuracy_value', 'NONE');
#13931=VERTEX_POINT ( 'NONE', #15040 ) ;
#14006=ORIENTED_EDGE ( 'NONE', *, *, #13422, .T. ) ;
#14018=CARTESIAN_POINT ( 'NONE',  ( 4.271534284832219323E-17, 3.369532131271296443E-15, 6.999999999999989342 ) ) ;
#14077=DIRECTION ( 'NONE',  ( -0.9237280213470681067, -0.3830490080632377725, 0.000000000000000000 ) ) ;
#14102=CIRCLE ( 'NONE', #6747, 3.799999999999999378 ) ;
#14132=DIRECTION ( 'NONE',  ( 0.000000000000000000, 0.000000000000000000, 1.000000000000000000 ) ) ;
#14141=VERTEX_POINT ( 'NONE', #7496 ) ;
#14154=EDGE_CURVE ( 'NONE', #12618, #11359, #12165, .T. ) ;
#14174=CIRCLE ( 'NONE', #3615, 4.000000000000000888 ) ;
#14176=COLOUR_RGB ( '',0.8941176470588234615, 0.8941176470588234615, 0.8941176470588234615 ) ;
#14259=EDGE_CURVE ( 'NONE', #4276, #3346, #3147, .T. ) ;
#14261=DIRECTION ( 'NONE',  ( 0.000000000000000000, 0.000000000000000000, 1.000000000000000000 ) ) ;
#14337=VECTOR ( 'NONE', #8854, 1000.000000000000000 ) ;
#14351=AXIS2_PLACEMENT_3D ( 'NONE', #5469, #9991, #13757 ) ;
#14383=CARTESIAN_POINT ( 'NONE',  ( 3.510166481118872639, 1.455586230640303791, -7.800000000000008704 ) ) ;
#14417=DIRECTION ( 'NONE',  ( -0.000000000000000000, -0.000000000000000000, -1.000000000000000000 ) ) ;
#14448=CARTESIAN_POINT ( 'NONE',  ( -4.000000000000000888, 0.000000000000000000, -7.800000000000010481 ) ) ;
#14483=ORIENTED_EDGE ( 'NONE', *, *, #8037, .T. ) ;
#14487=DIRECTION ( 'NONE',  ( -0.9237280213470681067, -0.3830490080632377725, 0.000000000000000000 ) ) ;
#14516=DIRECTION ( 'NONE',  ( 1.000000000000000000, 0.000000000000000000, 0.000000000000000000 ) ) ;
#14580=ORIENTED_EDGE ( 'NONE', *, *, #13512, .F. ) ;
#14593=LINE ( 'NONE', #12282, #5805 ) ;
#14625=ORIENTED_EDGE ( 'NONE', *, *, #7762, .T. ) ;
#14662=ORIENTED_EDGE ( 'NONE', *, *, #14894, .F. ) ;
#14674=CARTESIAN_POINT ( 'NONE',  ( 0.000000000000000000, 0.000000000000000000, -10.00000000000000000 ) ) ;
#14677=DIRECTION ( 'NONE',  ( -5.339417856040273846E-17, -1.063174570779084847E-17, 1.000000000000000000 ) ) ;
#14688=ORIENTED_EDGE ( 'NONE', *, *, #1569, .T. ) ;
#14791=LINE ( 'NONE', #2955, #10672 ) ;
#14835=ADVANCED_FACE ( 'NONE', ( #577 ), #5296, .T. ) ;
#14867=ORIENTED_EDGE ( 'NONE', *, *, #13512, .T. ) ;
#14886=EDGE_CURVE ( 'NONE', #3346, #4276, #6069, .T. ) ;
#14894=EDGE_CURVE ( 'NONE', #6657, #13931, #1157, .T. ) ;
#14904=EDGE_LOOP ( 'NONE', ( #9253, #14006, #7531, #14909 ) ) ;
#14909=ORIENTED_EDGE ( 'NONE', *, *, #6559, .F. ) ;
#14910=AXIS2_PLACEMENT_3D ( 'NONE', #5220, #8585, #2820 ) ;
#14941=AXIS2_PLACEMENT_3D ( 'NONE', #8693, #14132, #11465 ) ;
#14944=FACE_OUTER_BOUND ( 'NONE', #13753, .T. ) ;
#14983=ADVANCED_BREP_SHAPE_REPRESENTATION ( '', ( #3717, #1376 ), #12207 ) ;
#15029=LINE ( 'NONE', #2414, #8556 ) ;
#15040=CARTESIAN_POINT ( 'NONE',  ( -4.000000000000000888, 0.000000000000000000, -10.00000000000000000 ) ) ;
#15058=FACE_OUTER_BOUND ( 'NONE', #5650, .T. ) ;
#15074=CARTESIAN_POINT ( 'NONE',  ( 0.000000000000000000, 0.000000000000000000, 6.999999999999989342 ) ) ;
#15081=DIRECTION ( 'NONE',  ( -1.000000000000000000, 0.000000000000000000, 0.000000000000000000 ) ) ;
#15097=EDGE_CURVE ( 'NONE', #9762, #10385, #7055, .T. ) ;
#15107=ORIENTED_EDGE ( 'NONE', *, *, #15097, .T. ) ;
#15108=PLANE ( 'NONE',  #8167 ) ;
#15280=COLOUR_RGB('Off White',0.89,0.88,0.83);
#15281=FILL_AREA_STYLE_COLOUR('',#15280);
#15282=FILL_AREA_STYLE('',(#15281));
#15283=SURFACE_STYLE_FILL_AREA(#15282);
#15284=SURFACE_SIDE_STYLE('',(#15283));
#15285=SURFACE_STYLE_USAGE(.BOTH.,#15284);
#15286=PRESENTATION_STYLE_ASSIGNMENT((#15285));
ENDSEC;
END-ISO-10303-21;
